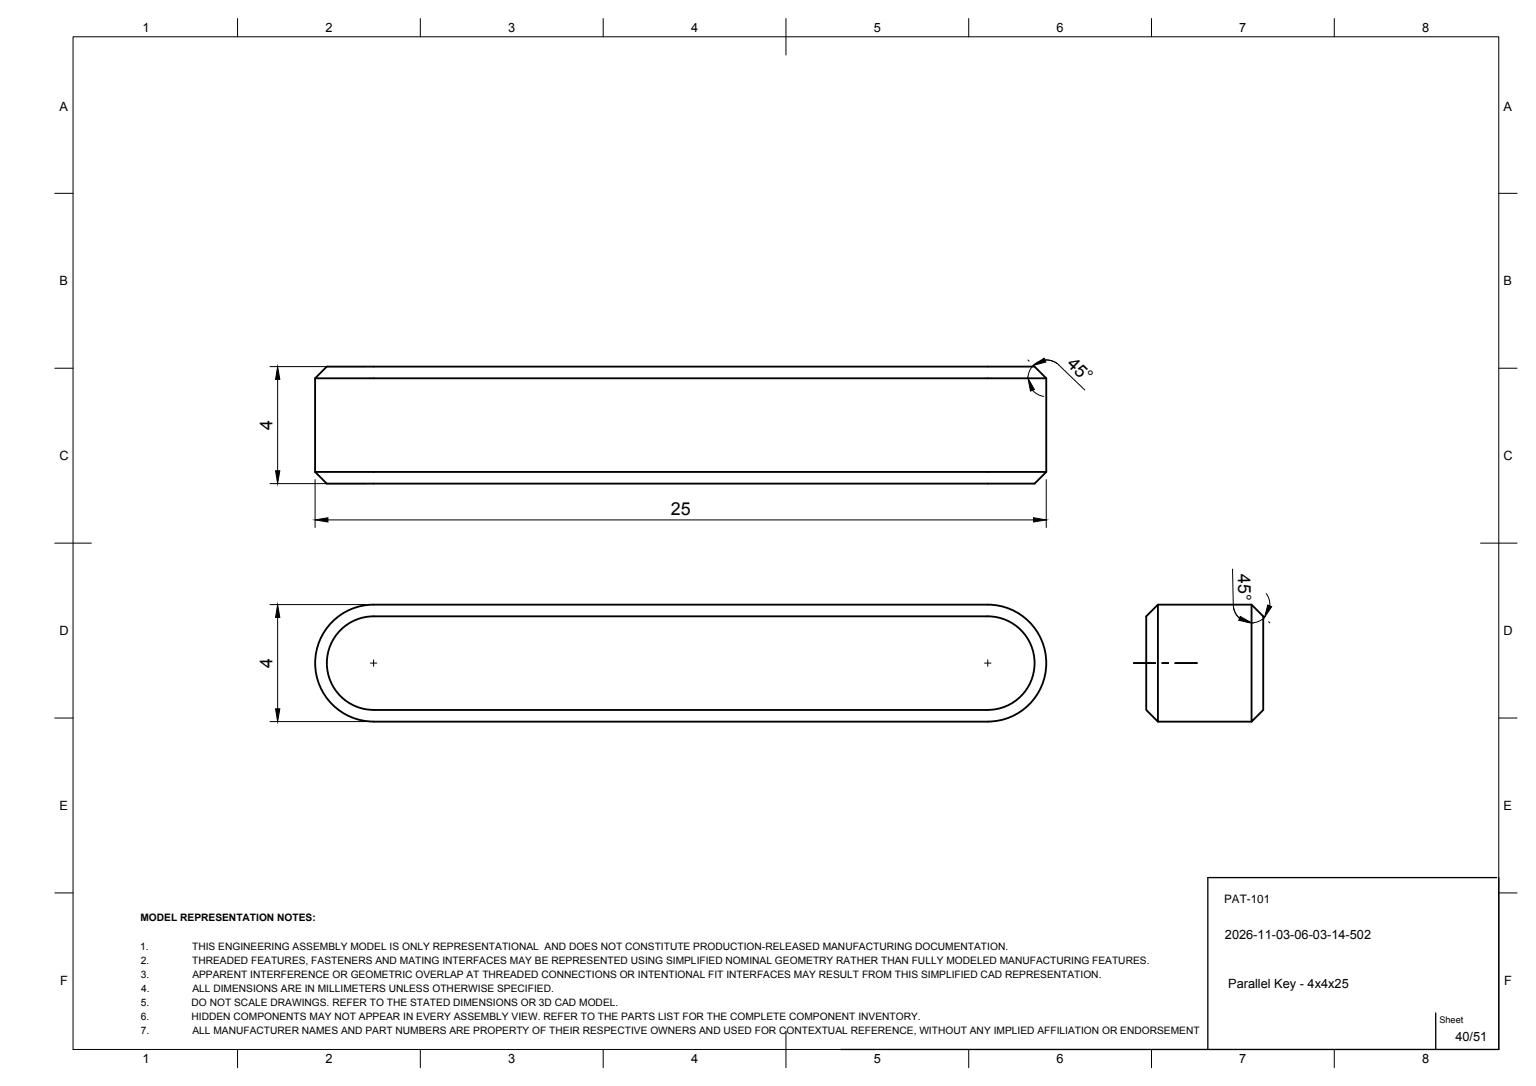
ISO-10303-21;
HEADER;
/* Generated by software containing ST-Developer
 * from STEP Tools, Inc. (www.steptools.com) 
 */

FILE_DESCRIPTION(
/* description */ ('Spur gear reduction stage 2-1 on bearing plates'),
/* implementation_level */ '2;1');

FILE_NAME(
/* name */ 'Parallel Key - 4x4x25.step',
/* time_stamp */ '2026-10-28T03:22:07-07:00',
/* author */ (''),
/* organization */ (''),
/* preprocessor_version */ 'ST-DEVELOPER v20.2',
/* originating_system */ 'Autodesk Translation Framework v15.17.0.0',
/* authorisation */ '');

FILE_SCHEMA (('AUTOMOTIVE_DESIGN { 1 0 10303 214 3 1 1 }'));
ENDSEC;

DATA;
#10=MECHANICAL_DESIGN_GEOMETRIC_PRESENTATION_REPRESENTATION('',(#994),#53909);
#852=CONICAL_SURFACE('',#12655,0.18,0.785398163397448);
#853=CONICAL_SURFACE('',#12659,0.18,0.785398163397448);
#854=CONICAL_SURFACE('',#12667,0.18,0.785398163397449);
#855=CONICAL_SURFACE('',#12670,0.18,0.785398163397449);
#893=SHAPE_REPRESENTATION_RELATIONSHIP('SRR','None',#54123,#936);
#936=ADVANCED_BREP_SHAPE_REPRESENTATION('',(#1049),#53897);
#994=STYLED_ITEM('',(#54397),#1049);
#1049=MANIFOLD_SOLID_BREP('Body1',#11321);
#1407=PLANE('',#12654);
#1408=PLANE('',#12658);
#1409=PLANE('',#12664);
#1410=PLANE('',#12665);
#1411=PLANE('',#12666);
#1412=PLANE('',#12669);
#1413=PLANE('',#12674);
#1414=PLANE('',#12675);
#1909=FACE_OUTER_BOUND('',#2714,.T.);
#1910=FACE_OUTER_BOUND('',#2715,.T.);
#1911=FACE_OUTER_BOUND('',#2716,.T.);
#1912=FACE_OUTER_BOUND('',#2717,.T.);
#1913=FACE_OUTER_BOUND('',#2718,.T.);
#1914=FACE_OUTER_BOUND('',#2719,.T.);
#1915=FACE_OUTER_BOUND('',#2720,.T.);
#1916=FACE_OUTER_BOUND('',#2721,.T.);
#1917=FACE_OUTER_BOUND('',#2722,.T.);
#1918=FACE_OUTER_BOUND('',#2723,.T.);
#1919=FACE_OUTER_BOUND('',#2724,.T.);
#1920=FACE_OUTER_BOUND('',#2725,.T.);
#1921=FACE_OUTER_BOUND('',#2726,.T.);
#1922=FACE_OUTER_BOUND('',#2727,.T.);
#2714=EDGE_LOOP('',(#9134,#9135,#9136,#9137));
#2715=EDGE_LOOP('',(#9138,#9139,#9140,#9141));
#2716=EDGE_LOOP('',(#9142,#9143,#9144,#9145));
#2717=EDGE_LOOP('',(#9146,#9147,#9148,#9149));
#2718=EDGE_LOOP('',(#9150,#9151,#9152,#9153));
#2719=EDGE_LOOP('',(#9154,#9155,#9156,#9157));
#2720=EDGE_LOOP('',(#9158,#9159,#9160,#9161));
#2721=EDGE_LOOP('',(#9162,#9163,#9164,#9165));
#2722=EDGE_LOOP('',(#9166,#9167,#9168,#9169));
#2723=EDGE_LOOP('',(#9170,#9171,#9172,#9173));
#2724=EDGE_LOOP('',(#9174,#9175,#9176,#9177));
#2725=EDGE_LOOP('',(#9178,#9179,#9180,#9181));
#2726=EDGE_LOOP('',(#9182,#9183,#9184,#9185));
#2727=EDGE_LOOP('',(#9186,#9187,#9188,#9189));
#3353=LINE('',#29786,#3994);
#3354=LINE('',#29788,#3995);
#3355=LINE('',#29790,#3996);
#3356=LINE('',#29791,#3997);
#3357=LINE('',#29795,#3998);
#3358=LINE('',#29801,#3999);
#3359=LINE('',#29802,#4000);
#3360=LINE('',#29803,#4001);
#3361=LINE('',#29809,#4002);
#3362=LINE('',#29812,#4003);
#3363=LINE('',#29815,#4004);
#3364=LINE('',#29816,#4005);
#3365=LINE('',#29820,#4006);
#3366=LINE('',#29822,#4007);
#3367=LINE('',#29823,#4008);
#3368=LINE('',#29826,#4009);
#3369=LINE('',#29831,#4010);
#3370=LINE('',#29832,#4011);
#3371=LINE('',#29833,#4012);
#3372=LINE('',#29838,#4013);
#3994=VECTOR('',#15056,1.);
#3995=VECTOR('',#15057,1.);
#3996=VECTOR('',#15058,1.);
#3997=VECTOR('',#15059,1.);
#3998=VECTOR('',#15062,1.);
#3999=VECTOR('',#15069,1.);
#4000=VECTOR('',#15070,1.);
#4001=VECTOR('',#15071,1.);
#4002=VECTOR('',#15080,1.);
#4003=VECTOR('',#15083,1.);
#4004=VECTOR('',#15086,1.);
#4005=VECTOR('',#15087,1.);
#4006=VECTOR('',#15092,1.);
#4007=VECTOR('',#15093,1.);
#4008=VECTOR('',#15094,1.);
#4009=VECTOR('',#15097,1.);
#4010=VECTOR('',#15102,1.);
#4011=VECTOR('',#15103,1.);
#4012=VECTOR('',#15104,1.);
#4013=VECTOR('',#15113,1.);
#4654=CIRCLE('',#12656,0.16);
#4655=CIRCLE('',#12657,0.2);
#4656=CIRCLE('',#12660,0.16);
#4657=CIRCLE('',#12661,0.2);
#4658=CIRCLE('',#12663,0.2);
#4659=CIRCLE('',#12668,0.16);
#4660=CIRCLE('',#12671,0.2);
#4661=CIRCLE('',#12672,0.16);
#5392=VERTEX_POINT('',#29784);
#5393=VERTEX_POINT('',#29785);
#5394=VERTEX_POINT('',#29787);
#5395=VERTEX_POINT('',#29789);
#5396=VERTEX_POINT('',#29793);
#5397=VERTEX_POINT('',#29794);
#5398=VERTEX_POINT('',#29799);
#5399=VERTEX_POINT('',#29800);
#5400=VERTEX_POINT('',#29808);
#5401=VERTEX_POINT('',#29810);
#5402=VERTEX_POINT('',#29814);
#5403=VERTEX_POINT('',#29819);
#5404=VERTEX_POINT('',#29821);
#5405=VERTEX_POINT('',#29825);
#5406=VERTEX_POINT('',#29829);
#5407=VERTEX_POINT('',#29830);
#6709=EDGE_CURVE('',#5392,#5393,#3353,.T.);
#6710=EDGE_CURVE('',#5393,#5394,#3354,.T.);
#6711=EDGE_CURVE('',#5394,#5395,#3355,.T.);
#6712=EDGE_CURVE('',#5395,#5392,#3356,.T.);
#6713=EDGE_CURVE('',#5396,#5397,#3357,.T.);
#6714=EDGE_CURVE('',#5397,#5393,#4654,.T.);
#6715=EDGE_CURVE('',#5392,#5396,#4655,.T.);
#6716=EDGE_CURVE('',#5398,#5399,#3358,.T.);
#6717=EDGE_CURVE('',#5399,#5397,#3359,.T.);
#6718=EDGE_CURVE('',#5396,#5398,#3360,.T.);
#6719=EDGE_CURVE('',#5394,#5399,#4656,.T.);
#6720=EDGE_CURVE('',#5398,#5395,#4657,.T.);
#6721=EDGE_CURVE('',#5400,#5392,#3361,.T.);
#6722=EDGE_CURVE('',#5401,#5400,#4658,.T.);
#6723=EDGE_CURVE('',#5401,#5396,#3362,.T.);
#6724=EDGE_CURVE('',#5402,#5395,#3363,.T.);
#6725=EDGE_CURVE('',#5400,#5402,#3364,.T.);
#6726=EDGE_CURVE('',#5403,#5400,#3365,.T.);
#6727=EDGE_CURVE('',#5402,#5404,#3366,.T.);
#6728=EDGE_CURVE('',#5404,#5403,#3367,.T.);
#6729=EDGE_CURVE('',#5405,#5401,#3368,.T.);
#6730=EDGE_CURVE('',#5403,#5405,#4659,.T.);
#6731=EDGE_CURVE('',#5406,#5407,#3369,.T.);
#6732=EDGE_CURVE('',#5407,#5401,#3370,.T.);
#6733=EDGE_CURVE('',#5405,#5406,#3371,.T.);
#6734=EDGE_CURVE('',#5402,#5407,#4660,.T.);
#6735=EDGE_CURVE('',#5406,#5404,#4661,.T.);
#6736=EDGE_CURVE('',#5407,#5398,#3372,.T.);
#9134=ORIENTED_EDGE('',*,*,#6709,.T.);
#9135=ORIENTED_EDGE('',*,*,#6710,.T.);
#9136=ORIENTED_EDGE('',*,*,#6711,.T.);
#9137=ORIENTED_EDGE('',*,*,#6712,.T.);
#9138=ORIENTED_EDGE('',*,*,#6713,.T.);
#9139=ORIENTED_EDGE('',*,*,#6714,.T.);
#9140=ORIENTED_EDGE('',*,*,#6709,.F.);
#9141=ORIENTED_EDGE('',*,*,#6715,.T.);
#9142=ORIENTED_EDGE('',*,*,#6716,.T.);
#9143=ORIENTED_EDGE('',*,*,#6717,.T.);
#9144=ORIENTED_EDGE('',*,*,#6713,.F.);
#9145=ORIENTED_EDGE('',*,*,#6718,.T.);
#9146=ORIENTED_EDGE('',*,*,#6711,.F.);
#9147=ORIENTED_EDGE('',*,*,#6719,.T.);
#9148=ORIENTED_EDGE('',*,*,#6716,.F.);
#9149=ORIENTED_EDGE('',*,*,#6720,.T.);
#9150=ORIENTED_EDGE('',*,*,#6715,.F.);
#9151=ORIENTED_EDGE('',*,*,#6721,.F.);
#9152=ORIENTED_EDGE('',*,*,#6722,.F.);
#9153=ORIENTED_EDGE('',*,*,#6723,.T.);
#9154=ORIENTED_EDGE('',*,*,#6712,.F.);
#9155=ORIENTED_EDGE('',*,*,#6724,.F.);
#9156=ORIENTED_EDGE('',*,*,#6725,.F.);
#9157=ORIENTED_EDGE('',*,*,#6721,.T.);
#9158=ORIENTED_EDGE('',*,*,#6710,.F.);
#9159=ORIENTED_EDGE('',*,*,#6714,.F.);
#9160=ORIENTED_EDGE('',*,*,#6717,.F.);
#9161=ORIENTED_EDGE('',*,*,#6719,.F.);
#9162=ORIENTED_EDGE('',*,*,#6726,.T.);
#9163=ORIENTED_EDGE('',*,*,#6725,.T.);
#9164=ORIENTED_EDGE('',*,*,#6727,.T.);
#9165=ORIENTED_EDGE('',*,*,#6728,.T.);
#9166=ORIENTED_EDGE('',*,*,#6729,.T.);
#9167=ORIENTED_EDGE('',*,*,#6722,.T.);
#9168=ORIENTED_EDGE('',*,*,#6726,.F.);
#9169=ORIENTED_EDGE('',*,*,#6730,.T.);
#9170=ORIENTED_EDGE('',*,*,#6731,.T.);
#9171=ORIENTED_EDGE('',*,*,#6732,.T.);
#9172=ORIENTED_EDGE('',*,*,#6729,.F.);
#9173=ORIENTED_EDGE('',*,*,#6733,.T.);
#9174=ORIENTED_EDGE('',*,*,#6727,.F.);
#9175=ORIENTED_EDGE('',*,*,#6734,.T.);
#9176=ORIENTED_EDGE('',*,*,#6731,.F.);
#9177=ORIENTED_EDGE('',*,*,#6735,.T.);
#9178=ORIENTED_EDGE('',*,*,#6720,.F.);
#9179=ORIENTED_EDGE('',*,*,#6736,.F.);
#9180=ORIENTED_EDGE('',*,*,#6734,.F.);
#9181=ORIENTED_EDGE('',*,*,#6724,.T.);
#9182=ORIENTED_EDGE('',*,*,#6728,.F.);
#9183=ORIENTED_EDGE('',*,*,#6735,.F.);
#9184=ORIENTED_EDGE('',*,*,#6733,.F.);
#9185=ORIENTED_EDGE('',*,*,#6730,.F.);
#9186=ORIENTED_EDGE('',*,*,#6718,.F.);
#9187=ORIENTED_EDGE('',*,*,#6723,.F.);
#9188=ORIENTED_EDGE('',*,*,#6732,.F.);
#9189=ORIENTED_EDGE('',*,*,#6736,.T.);
#10563=CYLINDRICAL_SURFACE('',#12662,0.2);
#10564=CYLINDRICAL_SURFACE('',#12673,0.2);
#11029=ADVANCED_FACE('',(#1909),#1407,.T.);
#11030=ADVANCED_FACE('',(#1910),#852,.T.);
#11031=ADVANCED_FACE('',(#1911),#1408,.T.);
#11032=ADVANCED_FACE('',(#1912),#853,.T.);
#11033=ADVANCED_FACE('',(#1913),#10563,.T.);
#11034=ADVANCED_FACE('',(#1914),#1409,.T.);
#11035=ADVANCED_FACE('',(#1915),#1410,.T.);
#11036=ADVANCED_FACE('',(#1916),#1411,.T.);
#11037=ADVANCED_FACE('',(#1917),#854,.T.);
#11038=ADVANCED_FACE('',(#1918),#1412,.T.);
#11039=ADVANCED_FACE('',(#1919),#855,.T.);
#11040=ADVANCED_FACE('',(#1920),#10564,.T.);
#11041=ADVANCED_FACE('',(#1921),#1413,.F.);
#11042=ADVANCED_FACE('',(#1922),#1414,.T.);
#11321=CLOSED_SHELL('',(#11029,#11030,#11031,#11032,#11033,#11034,#11035,
#11036,#11037,#11038,#11039,#11040,#11041,#11042));
#12653=AXIS2_PLACEMENT_3D('',#29782,#15052,#15053);
#12654=AXIS2_PLACEMENT_3D('',#29783,#15054,#15055);
#12655=AXIS2_PLACEMENT_3D('',#29792,#15060,#15061);
#12656=AXIS2_PLACEMENT_3D('',#29796,#15063,#15064);
#12657=AXIS2_PLACEMENT_3D('',#29797,#15065,#15066);
#12658=AXIS2_PLACEMENT_3D('',#29798,#15067,#15068);
#12659=AXIS2_PLACEMENT_3D('',#29804,#15072,#15073);
#12660=AXIS2_PLACEMENT_3D('',#29805,#15074,#15075);
#12661=AXIS2_PLACEMENT_3D('',#29806,#15076,#15077);
#12662=AXIS2_PLACEMENT_3D('',#29807,#15078,#15079);
#12663=AXIS2_PLACEMENT_3D('',#29811,#15081,#15082);
#12664=AXIS2_PLACEMENT_3D('',#29813,#15084,#15085);
#12665=AXIS2_PLACEMENT_3D('',#29817,#15088,#15089);
#12666=AXIS2_PLACEMENT_3D('',#29818,#15090,#15091);
#12667=AXIS2_PLACEMENT_3D('',#29824,#15095,#15096);
#12668=AXIS2_PLACEMENT_3D('',#29827,#15098,#15099);
#12669=AXIS2_PLACEMENT_3D('',#29828,#15100,#15101);
#12670=AXIS2_PLACEMENT_3D('',#29834,#15105,#15106);
#12671=AXIS2_PLACEMENT_3D('',#29835,#15107,#15108);
#12672=AXIS2_PLACEMENT_3D('',#29836,#15109,#15110);
#12673=AXIS2_PLACEMENT_3D('',#29837,#15111,#15112);
#12674=AXIS2_PLACEMENT_3D('',#29839,#15114,#15115);
#12675=AXIS2_PLACEMENT_3D('',#29840,#15116,#15117);
#15052=DIRECTION('axis',(0.,0.,1.));
#15053=DIRECTION('refdir',(1.,0.,0.));
#15054=DIRECTION('center_axis',(0.,0.707106781186548,0.707106781186547));
#15055=DIRECTION('ref_axis',(1.,0.,0.));
#15056=DIRECTION('',(-3.92523114670944E-15,-0.707106781186547,0.707106781186548));
#15057=DIRECTION('',(1.,0.,0.));
#15058=DIRECTION('',(0.,0.707106781186547,-0.707106781186548));
#15059=DIRECTION('',(-1.,0.,0.));
#15060=DIRECTION('center_axis',(0.,0.,-1.));
#15061=DIRECTION('ref_axis',(0.,1.,0.));
#15062=DIRECTION('',(0.,0.707106781186548,0.707106781186548));
#15063=DIRECTION('center_axis',(0.,0.,-1.));
#15064=DIRECTION('ref_axis',(0.,1.,0.));
#15065=DIRECTION('center_axis',(0.,0.,1.));
#15066=DIRECTION('ref_axis',(0.,1.,0.));
#15067=DIRECTION('center_axis',(0.,-0.707106781186548,0.707106781186547));
#15068=DIRECTION('ref_axis',(1.,0.,0.));
#15069=DIRECTION('',(3.92523114670944E-15,0.707106781186547,0.707106781186548));
#15070=DIRECTION('',(-1.,0.,0.));
#15071=DIRECTION('',(1.,0.,0.));
#15072=DIRECTION('center_axis',(0.,0.,-1.));
#15073=DIRECTION('ref_axis',(0.,-1.,0.));
#15074=DIRECTION('center_axis',(0.,0.,-1.));
#15075=DIRECTION('ref_axis',(0.,-1.,0.));
#15076=DIRECTION('center_axis',(0.,0.,1.));
#15077=DIRECTION('ref_axis',(0.,-1.,0.));
#15078=DIRECTION('center_axis',(0.,0.,1.));
#15079=DIRECTION('ref_axis',(0.,1.,0.));
#15080=DIRECTION('',(0.,0.,1.));
#15081=DIRECTION('center_axis',(0.,0.,-1.));
#15082=DIRECTION('ref_axis',(0.,1.,0.));
#15083=DIRECTION('',(0.,0.,1.));
#15084=DIRECTION('center_axis',(0.,1.,0.));
#15085=DIRECTION('ref_axis',(-1.,0.,0.));
#15086=DIRECTION('',(0.,0.,1.));
#15087=DIRECTION('',(1.,0.,0.));
#15088=DIRECTION('center_axis',(0.,0.,1.));
#15089=DIRECTION('ref_axis',(1.,0.,0.));
#15090=DIRECTION('center_axis',(0.,0.707106781186548,-0.707106781186548));
#15091=DIRECTION('ref_axis',(-1.,0.,0.));
#15092=DIRECTION('',(3.92523114670944E-15,0.707106781186548,0.707106781186548));
#15093=DIRECTION('',(0.,-0.707106781186548,-0.707106781186548));
#15094=DIRECTION('',(-1.,0.,0.));
#15095=DIRECTION('center_axis',(0.,0.,1.));
#15096=DIRECTION('ref_axis',(0.,1.,0.));
#15097=DIRECTION('',(0.,-0.707106781186548,0.707106781186547));
#15098=DIRECTION('center_axis',(0.,0.,1.));
#15099=DIRECTION('ref_axis',(0.,1.,0.));
#15100=DIRECTION('center_axis',(0.,-0.707106781186548,-0.707106781186548));
#15101=DIRECTION('ref_axis',(-1.,0.,0.));
#15102=DIRECTION('',(-3.92523114670944E-15,-0.707106781186548,0.707106781186548));
#15103=DIRECTION('',(-1.,0.,0.));
#15104=DIRECTION('',(1.,0.,0.));
#15105=DIRECTION('center_axis',(0.,0.,1.));
#15106=DIRECTION('ref_axis',(0.,-1.,0.));
#15107=DIRECTION('center_axis',(0.,0.,-1.));
#15108=DIRECTION('ref_axis',(0.,-1.,0.));
#15109=DIRECTION('center_axis',(0.,0.,1.));
#15110=DIRECTION('ref_axis',(0.,-1.,0.));
#15111=DIRECTION('center_axis',(0.,0.,1.));
#15112=DIRECTION('ref_axis',(0.,-1.,0.));
#15113=DIRECTION('',(0.,0.,1.));
#15114=DIRECTION('center_axis',(0.,0.,1.));
#15115=DIRECTION('ref_axis',(1.,0.,0.));
#15116=DIRECTION('center_axis',(0.,-1.,0.));
#15117=DIRECTION('ref_axis',(1.,0.,0.));
#29782=CARTESIAN_POINT('',(0.,0.,0.));
#29783=CARTESIAN_POINT('Origin',(0.525,0.18,0.38));
#29784=CARTESIAN_POINT('',(-1.05,0.2,0.36));
#29785=CARTESIAN_POINT('',(-1.05,0.16,0.4));
#29786=CARTESIAN_POINT('',(-1.05,0.2,0.36));
#29787=CARTESIAN_POINT('',(1.05,0.16,0.4));
#29788=CARTESIAN_POINT('',(0.525,0.16,0.4));
#29789=CARTESIAN_POINT('',(1.05,0.2,0.36));
#29790=CARTESIAN_POINT('',(1.05,0.16,0.4));
#29791=CARTESIAN_POINT('',(0.525,0.2,0.36));
#29792=CARTESIAN_POINT('Origin',(-1.05,0.,0.38));
#29793=CARTESIAN_POINT('',(-1.05,-0.2,0.36));
#29794=CARTESIAN_POINT('',(-1.05,-0.16,0.4));
#29795=CARTESIAN_POINT('',(-1.05,-0.2,0.36));
#29796=CARTESIAN_POINT('Origin',(-1.05,0.,0.4));
#29797=CARTESIAN_POINT('Origin',(-1.05,0.,0.36));
#29798=CARTESIAN_POINT('Origin',(-0.525,-0.18,0.38));
#29799=CARTESIAN_POINT('',(1.05,-0.2,0.36));
#29800=CARTESIAN_POINT('',(1.05,-0.16,0.4));
#29801=CARTESIAN_POINT('',(1.05,-0.2,0.36));
#29802=CARTESIAN_POINT('',(-0.525,-0.16,0.4));
#29803=CARTESIAN_POINT('',(-0.525,-0.2,0.36));
#29804=CARTESIAN_POINT('Origin',(1.05,0.,0.38));
#29805=CARTESIAN_POINT('Origin',(1.05,0.,0.4));
#29806=CARTESIAN_POINT('Origin',(1.05,0.,0.36));
#29807=CARTESIAN_POINT('Origin',(-1.05,0.,0.));
#29808=CARTESIAN_POINT('',(-1.05,0.2,0.04));
#29809=CARTESIAN_POINT('',(-1.05,0.2,0.));
#29810=CARTESIAN_POINT('',(-1.05,-0.2,0.04));
#29811=CARTESIAN_POINT('Origin',(-1.05,0.,0.04));
#29812=CARTESIAN_POINT('',(-1.05,-0.2,0.));
#29813=CARTESIAN_POINT('Origin',(1.05,0.2,0.));
#29814=CARTESIAN_POINT('',(1.05,0.2,0.04));
#29815=CARTESIAN_POINT('',(1.05,0.2,0.));
#29816=CARTESIAN_POINT('',(0.525,0.2,0.04));
#29817=CARTESIAN_POINT('Origin',(0.,0.,0.4));
#29818=CARTESIAN_POINT('Origin',(0.525,0.18,0.02));
#29819=CARTESIAN_POINT('',(-1.05,0.16,0.));
#29820=CARTESIAN_POINT('',(-1.05,0.16,0.));
#29821=CARTESIAN_POINT('',(1.05,0.16,0.));
#29822=CARTESIAN_POINT('',(1.05,0.2,0.04));
#29823=CARTESIAN_POINT('',(0.525,0.16,0.));
#29824=CARTESIAN_POINT('Origin',(-1.05,0.,0.02));
#29825=CARTESIAN_POINT('',(-1.05,-0.16,0.));
#29826=CARTESIAN_POINT('',(-1.05,-0.16,0.));
#29827=CARTESIAN_POINT('Origin',(-1.05,0.,0.));
#29828=CARTESIAN_POINT('Origin',(-0.525,-0.18,0.02));
#29829=CARTESIAN_POINT('',(1.05,-0.16,0.));
#29830=CARTESIAN_POINT('',(1.05,-0.2,0.04));
#29831=CARTESIAN_POINT('',(1.05,-0.16,0.));
#29832=CARTESIAN_POINT('',(-0.525,-0.2,0.04));
#29833=CARTESIAN_POINT('',(-0.525,-0.16,0.));
#29834=CARTESIAN_POINT('Origin',(1.05,0.,0.02));
#29835=CARTESIAN_POINT('Origin',(1.05,0.,0.04));
#29836=CARTESIAN_POINT('Origin',(1.05,0.,0.));
#29837=CARTESIAN_POINT('Origin',(1.05,0.,0.));
#29838=CARTESIAN_POINT('',(1.05,-0.2,0.));
#29839=CARTESIAN_POINT('Origin',(0.,0.,0.));
#29840=CARTESIAN_POINT('Origin',(-1.05,-0.2,0.));
#53847=UNCERTAINTY_MEASURE_WITH_UNIT(LENGTH_MEASURE(0.001),#53910,
'DISTANCE_ACCURACY_VALUE',
'Maximum model space distance between geometric entities at asserted c
onnectivities');
#53859=UNCERTAINTY_MEASURE_WITH_UNIT(LENGTH_MEASURE(0.001),#53910,
'DISTANCE_ACCURACY_VALUE',
'Maximum model space distance between geometric entities at asserted c
onnectivities');
#53897=(
GEOMETRIC_REPRESENTATION_CONTEXT(3)
GLOBAL_UNCERTAINTY_ASSIGNED_CONTEXT((#53847))
GLOBAL_UNIT_ASSIGNED_CONTEXT((#53910,#53912,#53913))
REPRESENTATION_CONTEXT('','3D')
);
#53909=(
GEOMETRIC_REPRESENTATION_CONTEXT(3)
GLOBAL_UNCERTAINTY_ASSIGNED_CONTEXT((#53859))
GLOBAL_UNIT_ASSIGNED_CONTEXT((#53910,#53912,#53913))
REPRESENTATION_CONTEXT('','3D')
);
#53910=(
LENGTH_UNIT()
NAMED_UNIT(*)
SI_UNIT(.CENTI.,.METRE.)
);
#53912=(
NAMED_UNIT(*)
PLANE_ANGLE_UNIT()
SI_UNIT($,.RADIAN.)
);
#53913=(
NAMED_UNIT(*)
SI_UNIT($,.STERADIAN.)
SOLID_ANGLE_UNIT()
);
#53951=SHAPE_DEFINITION_REPRESENTATION(#54049,#54123);
#54049=PRODUCT_DEFINITION_SHAPE('',$,#54173);
#54123=SHAPE_REPRESENTATION('',(#12653),#53897);
#54135=PRODUCT_DEFINITION_CONTEXT('part definition',#54284,'design');
#54173=PRODUCT_DEFINITION('Parallel Key - 4x4x25',
'Parallel Key - 4x4x25',#54222,#54135);
#54222=PRODUCT_DEFINITION_FORMATION('',$,#54323);
#54284=APPLICATION_CONTEXT(
'Core Data for Automotive Mechanical Design Process');
#54285=PRODUCT_CONTEXT('part definition',#54284,'mechanical');
#54323=PRODUCT('Parallel Key - 4x4x25','Parallel Key - 4x4x25',
'Parallel Key - 4x4x25',(#54285));
#54391=COLOUR_RGB('Grey',0.48,0.52,0.57);
#54392=FILL_AREA_STYLE_COLOUR('',#54391);
#54393=FILL_AREA_STYLE('',(#54392));
#54394=SURFACE_STYLE_FILL_AREA(#54393);
#54395=SURFACE_SIDE_STYLE('',(#54394));
#54396=SURFACE_STYLE_USAGE(.BOTH.,#54395);
#54397=PRESENTATION_STYLE_ASSIGNMENT((#54396));
ENDSEC;
END-ISO-10303-21;
